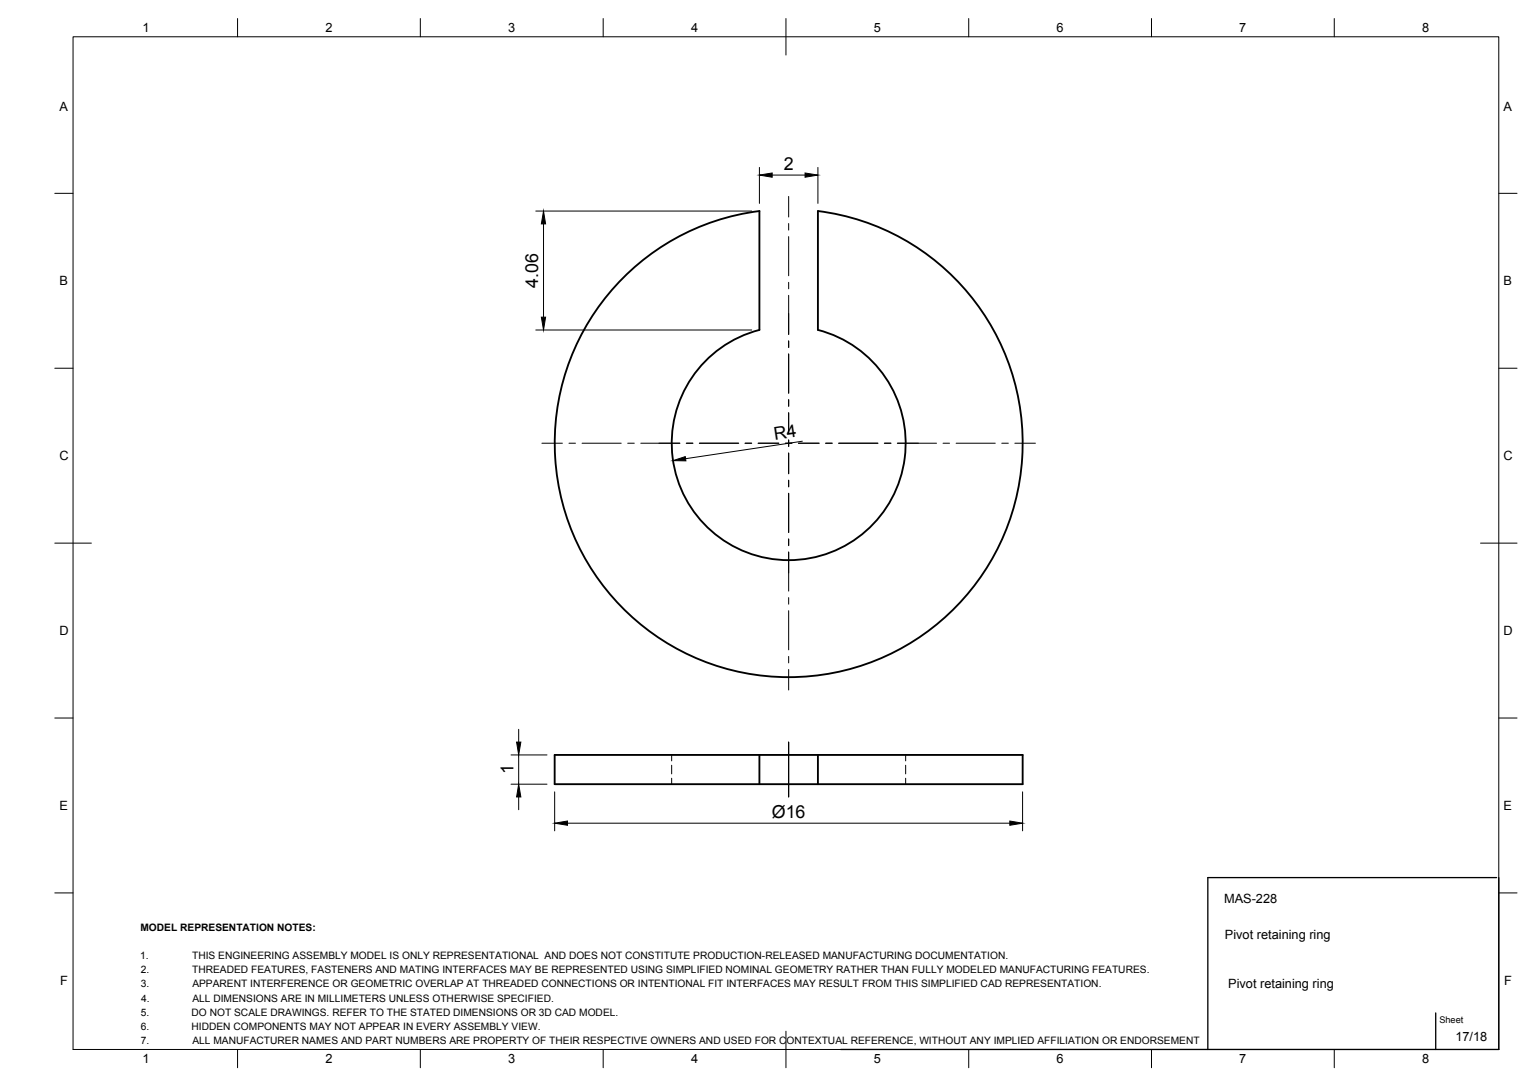
ISO-10303-21;
HEADER;
/* Generated by software containing ST-Developer
 * from STEP Tools, Inc. (www.steptools.com) 
 */

FILE_DESCRIPTION(
/* description */ ('Independent Peaucellier-Lipkin straight-line linkage. Radius arms 100
 mm, inversion-cell links 60 mm, crank radius and fixed-pivot spacing 
32 mm. Inversion constant 6400 mm squared, nominal output straight lin
e X=100 mm. Overhead bearing bridge clears the layered moving links. N
o accuracy or load rating assigned.'),
/* implementation_level */ '2;1');

FILE_NAME(
/* name */ 'Pivot retaining ring.step',
/* time_stamp */ '2026-11-09T18:06:16-08:00',
/* author */ (''),
/* organization */ (''),
/* preprocessor_version */ 'ST-DEVELOPER v20.2',
/* originating_system */ 'Autodesk Translation Framework v15.17.0.0',
/* authorisation */ '');

FILE_SCHEMA (('AUTOMOTIVE_DESIGN { 1 0 10303 214 3 1 1 }'));
ENDSEC;

DATA;
#10=MECHANICAL_DESIGN_GEOMETRIC_PRESENTATION_REPRESENTATION('',(#298),#3581);
#264=SHAPE_REPRESENTATION_RELATIONSHIP('SRR','None',#3698,#281);
#281=ADVANCED_BREP_SHAPE_REPRESENTATION('',(#315),#3580);
#298=STYLED_ITEM('',(#3787),#315);
#315=MANIFOLD_SOLID_BREP('Body1',#1884);
#421=PLANE('',#2290);
#422=PLANE('',#2291);
#423=PLANE('',#2292);
#424=PLANE('',#2299);
#530=FACE_OUTER_BOUND('',#689,.T.);
#531=FACE_OUTER_BOUND('',#690,.T.);
#532=FACE_OUTER_BOUND('',#691,.T.);
#533=FACE_OUTER_BOUND('',#692,.T.);
#534=FACE_OUTER_BOUND('',#693,.T.);
#535=FACE_OUTER_BOUND('',#694,.T.);
#689=EDGE_LOOP('',(#1684,#1685,#1686,#1687));
#690=EDGE_LOOP('',(#1688,#1689,#1690,#1691));
#691=EDGE_LOOP('',(#1692,#1693,#1694,#1695));
#692=EDGE_LOOP('',(#1696,#1697,#1698,#1699));
#693=EDGE_LOOP('',(#1700,#1701,#1702,#1703));
#694=EDGE_LOOP('',(#1704,#1705,#1706,#1707));
#785=LINE('',#3462,#883);
#786=LINE('',#3464,#884);
#787=LINE('',#3466,#885);
#788=LINE('',#3467,#886);
#789=LINE('',#3471,#887);
#790=LINE('',#3473,#888);
#791=LINE('',#3475,#889);
#792=LINE('',#3476,#890);
#883=VECTOR('',#2885,10.);
#884=VECTOR('',#2886,10.);
#885=VECTOR('',#2887,10.);
#886=VECTOR('',#2888,10.);
#887=VECTOR('',#2891,10.);
#888=VECTOR('',#2892,10.);
#889=VECTOR('',#2893,10.);
#890=VECTOR('',#2894,10.);
#985=CIRCLE('',#2293,8.);
#986=CIRCLE('',#2294,4.);
#987=CIRCLE('',#2296,4.);
#988=CIRCLE('',#2298,8.);
#1112=VERTEX_POINT('',#3460);
#1113=VERTEX_POINT('',#3461);
#1114=VERTEX_POINT('',#3463);
#1115=VERTEX_POINT('',#3465);
#1116=VERTEX_POINT('',#3469);
#1117=VERTEX_POINT('',#3470);
#1118=VERTEX_POINT('',#3472);
#1119=VERTEX_POINT('',#3474);
#1304=EDGE_CURVE('',#1112,#1113,#785,.T.);
#1305=EDGE_CURVE('',#1114,#1112,#786,.T.);
#1306=EDGE_CURVE('',#1115,#1114,#787,.T.);
#1307=EDGE_CURVE('',#1113,#1115,#788,.T.);
#1308=EDGE_CURVE('',#1116,#1117,#789,.T.);
#1309=EDGE_CURVE('',#1118,#1116,#790,.T.);
#1310=EDGE_CURVE('',#1119,#1118,#791,.T.);
#1311=EDGE_CURVE('',#1117,#1119,#792,.T.);
#1312=EDGE_CURVE('',#1114,#1119,#985,.T.);
#1313=EDGE_CURVE('',#1117,#1112,#986,.T.);
#1314=EDGE_CURVE('',#1116,#1113,#987,.T.);
#1315=EDGE_CURVE('',#1115,#1118,#988,.T.);
#1684=ORIENTED_EDGE('',*,*,#1304,.F.);
#1685=ORIENTED_EDGE('',*,*,#1305,.F.);
#1686=ORIENTED_EDGE('',*,*,#1306,.F.);
#1687=ORIENTED_EDGE('',*,*,#1307,.F.);
#1688=ORIENTED_EDGE('',*,*,#1308,.F.);
#1689=ORIENTED_EDGE('',*,*,#1309,.F.);
#1690=ORIENTED_EDGE('',*,*,#1310,.F.);
#1691=ORIENTED_EDGE('',*,*,#1311,.F.);
#1692=ORIENTED_EDGE('',*,*,#1311,.T.);
#1693=ORIENTED_EDGE('',*,*,#1312,.F.);
#1694=ORIENTED_EDGE('',*,*,#1305,.T.);
#1695=ORIENTED_EDGE('',*,*,#1313,.F.);
#1696=ORIENTED_EDGE('',*,*,#1308,.T.);
#1697=ORIENTED_EDGE('',*,*,#1313,.T.);
#1698=ORIENTED_EDGE('',*,*,#1304,.T.);
#1699=ORIENTED_EDGE('',*,*,#1314,.F.);
#1700=ORIENTED_EDGE('',*,*,#1310,.T.);
#1701=ORIENTED_EDGE('',*,*,#1315,.F.);
#1702=ORIENTED_EDGE('',*,*,#1306,.T.);
#1703=ORIENTED_EDGE('',*,*,#1312,.T.);
#1704=ORIENTED_EDGE('',*,*,#1309,.T.);
#1705=ORIENTED_EDGE('',*,*,#1314,.T.);
#1706=ORIENTED_EDGE('',*,*,#1307,.T.);
#1707=ORIENTED_EDGE('',*,*,#1315,.T.);
#1755=CYLINDRICAL_SURFACE('',#2295,4.);
#1756=CYLINDRICAL_SURFACE('',#2297,8.);
#1862=ADVANCED_FACE('',(#530),#421,.F.);
#1863=ADVANCED_FACE('',(#531),#422,.F.);
#1864=ADVANCED_FACE('',(#532),#423,.F.);
#1865=ADVANCED_FACE('',(#533),#1755,.F.);
#1866=ADVANCED_FACE('',(#534),#1756,.T.);
#1867=ADVANCED_FACE('',(#535),#424,.T.);
#1884=CLOSED_SHELL('',(#1862,#1863,#1864,#1865,#1866,#1867));
#2289=AXIS2_PLACEMENT_3D('',#3458,#2881,#2882);
#2290=AXIS2_PLACEMENT_3D('',#3459,#2883,#2884);
#2291=AXIS2_PLACEMENT_3D('',#3468,#2889,#2890);
#2292=AXIS2_PLACEMENT_3D('',#3477,#2895,#2896);
#2293=AXIS2_PLACEMENT_3D('',#3478,#2897,#2898);
#2294=AXIS2_PLACEMENT_3D('',#3479,#2899,#2900);
#2295=AXIS2_PLACEMENT_3D('',#3480,#2901,#2902);
#2296=AXIS2_PLACEMENT_3D('',#3481,#2903,#2904);
#2297=AXIS2_PLACEMENT_3D('',#3482,#2905,#2906);
#2298=AXIS2_PLACEMENT_3D('',#3483,#2907,#2908);
#2299=AXIS2_PLACEMENT_3D('',#3484,#2909,#2910);
#2881=DIRECTION('axis',(0.,0.,1.));
#2882=DIRECTION('refdir',(1.,0.,0.));
#2883=DIRECTION('center_axis',(-1.,0.,0.));
#2884=DIRECTION('ref_axis',(0.,1.,0.));
#2885=DIRECTION('',(0.,0.,1.));
#2886=DIRECTION('',(0.,-1.,0.));
#2887=DIRECTION('',(0.,0.,-1.));
#2888=DIRECTION('',(0.,1.,0.));
#2889=DIRECTION('center_axis',(1.,0.,0.));
#2890=DIRECTION('ref_axis',(0.,-1.,0.));
#2891=DIRECTION('',(0.,0.,-1.));
#2892=DIRECTION('',(0.,-1.,0.));
#2893=DIRECTION('',(0.,0.,1.));
#2894=DIRECTION('',(0.,1.,0.));
#2895=DIRECTION('center_axis',(0.,0.,1.));
#2896=DIRECTION('ref_axis',(1.,0.,0.));
#2897=DIRECTION('center_axis',(0.,0.,1.));
#2898=DIRECTION('ref_axis',(1.,0.,0.));
#2899=DIRECTION('center_axis',(0.,0.,-1.));
#2900=DIRECTION('ref_axis',(1.,0.,0.));
#2901=DIRECTION('center_axis',(0.,0.,1.));
#2902=DIRECTION('ref_axis',(6.12323399573677E-17,-1.,0.));
#2903=DIRECTION('center_axis',(0.,0.,-1.));
#2904=DIRECTION('ref_axis',(1.,0.,0.));
#2905=DIRECTION('center_axis',(0.,0.,1.));
#2906=DIRECTION('ref_axis',(6.12323399573677E-17,-1.,0.));
#2907=DIRECTION('center_axis',(0.,0.,1.));
#2908=DIRECTION('ref_axis',(1.,0.,0.));
#2909=DIRECTION('center_axis',(0.,0.,1.));
#2910=DIRECTION('ref_axis',(1.,0.,0.));
#3458=CARTESIAN_POINT('',(0.,0.,0.));
#3459=CARTESIAN_POINT('Origin',(-1.,0.,1.));
#3460=CARTESIAN_POINT('',(-1.,3.87298334620742,0.));
#3461=CARTESIAN_POINT('',(-1.,3.87298334620742,1.));
#3462=CARTESIAN_POINT('',(-1.,3.87298334620742,0.));
#3463=CARTESIAN_POINT('',(-1.,7.93725393319377,0.));
#3464=CARTESIAN_POINT('',(-1.,0.,0.));
#3465=CARTESIAN_POINT('',(-1.,7.93725393319377,1.));
#3466=CARTESIAN_POINT('',(-1.,7.93725393319377,0.));
#3467=CARTESIAN_POINT('',(-1.,0.,1.));
#3468=CARTESIAN_POINT('Origin',(1.,16.,1.));
#3469=CARTESIAN_POINT('',(1.,3.87298334620742,1.));
#3470=CARTESIAN_POINT('',(1.,3.87298334620742,0.));
#3471=CARTESIAN_POINT('',(1.,3.87298334620742,0.));
#3472=CARTESIAN_POINT('',(1.,7.93725393319377,1.));
#3473=CARTESIAN_POINT('',(1.,8.,1.));
#3474=CARTESIAN_POINT('',(1.,7.93725393319377,0.));
#3475=CARTESIAN_POINT('',(1.,7.93725393319377,0.));
#3476=CARTESIAN_POINT('',(1.,8.,0.));
#3477=CARTESIAN_POINT('Origin',(0.,0.,0.));
#3478=CARTESIAN_POINT('Origin',(0.,0.,0.));
#3479=CARTESIAN_POINT('Origin',(0.,0.,0.));
#3480=CARTESIAN_POINT('Origin',(0.,0.,0.));
#3481=CARTESIAN_POINT('Origin',(0.,0.,1.));
#3482=CARTESIAN_POINT('Origin',(0.,0.,0.));
#3483=CARTESIAN_POINT('Origin',(0.,0.,1.));
#3484=CARTESIAN_POINT('Origin',(0.,0.,1.));
#3561=UNCERTAINTY_MEASURE_WITH_UNIT(LENGTH_MEASURE(0.01),#3582,
'DISTANCE_ACCURACY_VALUE',
'Maximum model space distance between geometric entities at asserted c
onnectivities');
#3562=UNCERTAINTY_MEASURE_WITH_UNIT(LENGTH_MEASURE(0.01),#3582,
'DISTANCE_ACCURACY_VALUE',
'Maximum model space distance between geometric entities at asserted c
onnectivities');
#3580=(
GEOMETRIC_REPRESENTATION_CONTEXT(3)
GLOBAL_UNCERTAINTY_ASSIGNED_CONTEXT((#3561))
GLOBAL_UNIT_ASSIGNED_CONTEXT((#3582,#3584,#3585))
REPRESENTATION_CONTEXT('','3D')
);
#3581=(
GEOMETRIC_REPRESENTATION_CONTEXT(3)
GLOBAL_UNCERTAINTY_ASSIGNED_CONTEXT((#3562))
GLOBAL_UNIT_ASSIGNED_CONTEXT((#3582,#3584,#3585))
REPRESENTATION_CONTEXT('','3D')
);
#3582=(
LENGTH_UNIT()
NAMED_UNIT(*)
SI_UNIT(.MILLI.,.METRE.)
);
#3584=(
NAMED_UNIT(*)
PLANE_ANGLE_UNIT()
SI_UNIT($,.RADIAN.)
);
#3585=(
NAMED_UNIT(*)
SI_UNIT($,.STERADIAN.)
SOLID_ANGLE_UNIT()
);
#3603=SHAPE_DEFINITION_REPRESENTATION(#3621,#3698);
#3621=PRODUCT_DEFINITION_SHAPE('',$,#3717);
#3698=SHAPE_REPRESENTATION('',(#2289),#3580);
#3699=PRODUCT_DEFINITION_CONTEXT('part definition',#3755,'design');
#3717=PRODUCT_DEFINITION('Pivot retaining ring','Pivot retaining ring',
#3735,#3699);
#3735=PRODUCT_DEFINITION_FORMATION('',$,#3774);
#3755=APPLICATION_CONTEXT(
'Core Data for Automotive Mechanical Design Process');
#3756=PRODUCT_CONTEXT('part definition',#3755,'mechanical');
#3774=PRODUCT('Pivot retaining ring','Pivot retaining ring',$,(#3756));
#3787=PRESENTATION_STYLE_ASSIGNMENT((#3800));
#3800=SURFACE_STYLE_USAGE(.BOTH.,#3813);
#3813=SURFACE_SIDE_STYLE('',(#3826));
#3826=SURFACE_STYLE_FILL_AREA(#3839);
#3839=FILL_AREA_STYLE('Dark gray',(#3852));
#3852=FILL_AREA_STYLE_COLOUR('Dark gray',#3865);
#3865=COLOUR_RGB('Dark gray',0.250980392156863,0.282352941176471,0.32156862745098);
ENDSEC;
END-ISO-10303-21;
